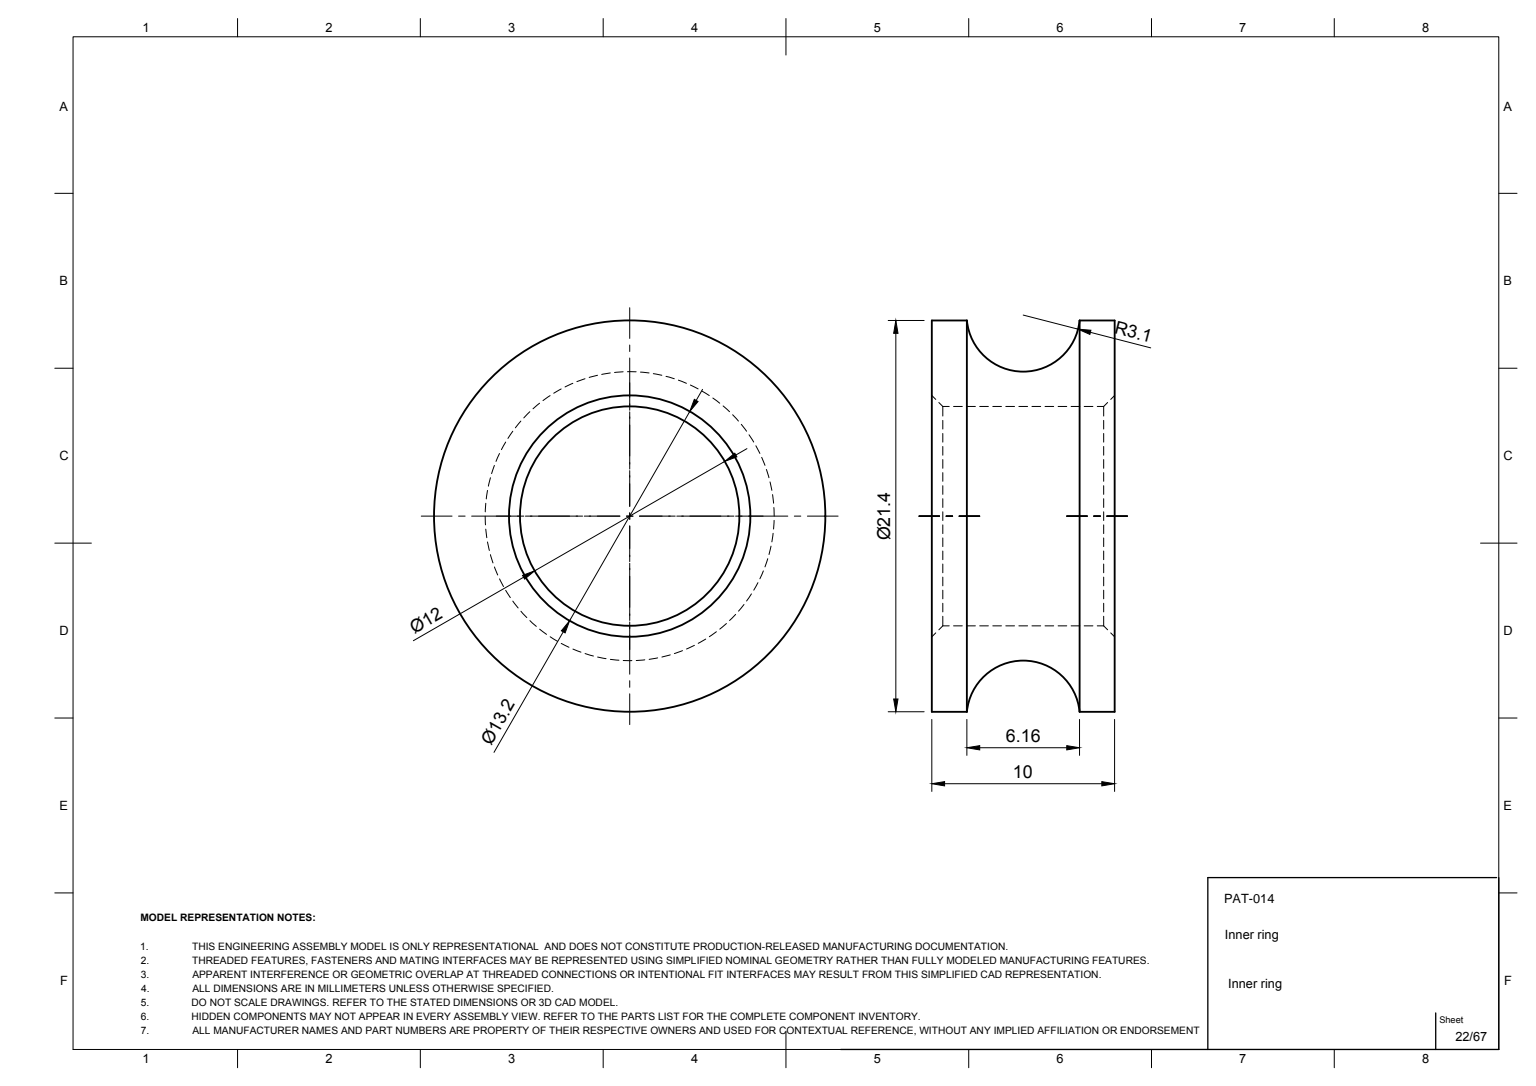
ISO-10303-21;
HEADER;
/* Generated by software containing ST-Developer
 * from STEP Tools, Inc. (www.steptools.com) 
 */

FILE_DESCRIPTION(
/* description */ ('Bin tilter linkage'),
/* implementation_level */ '2;1');

FILE_NAME(
/* name */ 'Inner ring.step',
/* time_stamp */ '2026-10-28T03:26:24-07:00',
/* author */ (''),
/* organization */ (''),
/* preprocessor_version */ 'ST-DEVELOPER v20.2',
/* originating_system */ 'Autodesk Translation Framework v15.17.0.0',
/* authorisation */ '');

FILE_SCHEMA (('AUTOMOTIVE_DESIGN { 1 0 10303 214 3 1 1 }'));
ENDSEC;

DATA;
#10=MECHANICAL_DESIGN_GEOMETRIC_PRESENTATION_REPRESENTATION('',(#934),#23728);
#627=TOROIDAL_SURFACE('',#14775,1.1,0.309556);
#636=CONICAL_SURFACE('',#14786,0.63,0.785398163397448);
#637=CONICAL_SURFACE('',#14793,0.63,0.785398163397448);
#722=SHAPE_REPRESENTATION_RELATIONSHIP('SRR','None',#24189,#828);
#828=ADVANCED_BREP_SHAPE_REPRESENTATION('',(#1047),#23689);
#934=STYLED_ITEM('',(#24765),#1047);
#1047=MANIFOLD_SOLID_BREP('Body1',#12465);
#1386=FACE_BOUND('',#3476,.T.);
#1387=FACE_BOUND('',#3479,.T.);
#1737=PLANE('',#14788);
#1738=PLANE('',#14791);
#2395=FACE_OUTER_BOUND('',#3471,.T.);
#2396=FACE_OUTER_BOUND('',#3472,.T.);
#2397=FACE_OUTER_BOUND('',#3473,.T.);
#2398=FACE_OUTER_BOUND('',#3474,.T.);
#2399=FACE_OUTER_BOUND('',#3475,.T.);
#2400=FACE_OUTER_BOUND('',#3477,.T.);
#2401=FACE_OUTER_BOUND('',#3478,.T.);
#2402=FACE_OUTER_BOUND('',#3480,.T.);
#3471=EDGE_LOOP('',(#10213,#10214,#10215,#10216,#10217,#10218));
#3472=EDGE_LOOP('',(#10219,#10220,#10221,#10222,#10223));
#3473=EDGE_LOOP('',(#10224,#10225,#10226,#10227));
#3474=EDGE_LOOP('',(#10228,#10229,#10230,#10231));
#3475=EDGE_LOOP('',(#10232));
#3476=EDGE_LOOP('',(#10233));
#3477=EDGE_LOOP('',(#10234,#10235,#10236,#10237,#10238));
#3478=EDGE_LOOP('',(#10239));
#3479=EDGE_LOOP('',(#10240));
#3480=EDGE_LOOP('',(#10241,#10242,#10243,#10244));
#4253=LINE('',#21872,#4928);
#4254=LINE('',#21878,#4929);
#4255=LINE('',#21882,#4930);
#4256=LINE('',#21888,#4931);
#4257=LINE('',#21893,#4932);
#4928=VECTOR('',#18090,1.070235);
#4929=VECTOR('',#18097,0.6);
#4930=VECTOR('',#18102,0.63);
#4931=VECTOR('',#18111,1.070235);
#4932=VECTOR('',#18118,0.63);
#5715=CIRCLE('',#14776,1.070235);
#5716=CIRCLE('',#14777,1.070235);
#5717=CIRCLE('',#14778,0.309556);
#5718=CIRCLE('',#14779,1.070235);
#5719=CIRCLE('',#14780,1.070235);
#5720=CIRCLE('',#14782,1.070235);
#5721=CIRCLE('',#14784,0.6);
#5722=CIRCLE('',#14785,0.6);
#5723=CIRCLE('',#14787,0.66);
#5724=CIRCLE('',#14790,1.070235);
#5725=CIRCLE('',#14792,0.66);
#6569=VERTEX_POINT('',#21861);
#6570=VERTEX_POINT('',#21862);
#6571=VERTEX_POINT('',#21865);
#6572=VERTEX_POINT('',#21867);
#6573=VERTEX_POINT('',#21871);
#6574=VERTEX_POINT('',#21875);
#6575=VERTEX_POINT('',#21877);
#6576=VERTEX_POINT('',#21881);
#6577=VERTEX_POINT('',#21886);
#6578=VERTEX_POINT('',#21890);
#7846=EDGE_CURVE('',#6569,#6570,#5715,.T.);
#7847=EDGE_CURVE('',#6570,#6569,#5716,.T.);
#7848=EDGE_CURVE('',#6570,#6571,#5717,.T.);
#7849=EDGE_CURVE('',#6572,#6571,#5718,.T.);
#7850=EDGE_CURVE('',#6571,#6572,#5719,.T.);
#7851=EDGE_CURVE('',#6572,#6573,#4253,.T.);
#7852=EDGE_CURVE('',#6573,#6573,#5720,.T.);
#7853=EDGE_CURVE('',#6574,#6574,#5721,.T.);
#7854=EDGE_CURVE('',#6574,#6575,#4254,.T.);
#7855=EDGE_CURVE('',#6575,#6575,#5722,.T.);
#7856=EDGE_CURVE('',#6575,#6576,#4255,.T.);
#7857=EDGE_CURVE('',#6576,#6576,#5723,.T.);
#7858=EDGE_CURVE('',#6577,#6577,#5724,.T.);
#7859=EDGE_CURVE('',#6577,#6569,#4256,.T.);
#7860=EDGE_CURVE('',#6578,#6578,#5725,.T.);
#7861=EDGE_CURVE('',#6578,#6574,#4257,.T.);
#10213=ORIENTED_EDGE('',*,*,#7846,.F.);
#10214=ORIENTED_EDGE('',*,*,#7847,.F.);
#10215=ORIENTED_EDGE('',*,*,#7848,.T.);
#10216=ORIENTED_EDGE('',*,*,#7849,.F.);
#10217=ORIENTED_EDGE('',*,*,#7850,.F.);
#10218=ORIENTED_EDGE('',*,*,#7848,.F.);
#10219=ORIENTED_EDGE('',*,*,#7849,.T.);
#10220=ORIENTED_EDGE('',*,*,#7850,.T.);
#10221=ORIENTED_EDGE('',*,*,#7851,.T.);
#10222=ORIENTED_EDGE('',*,*,#7852,.T.);
#10223=ORIENTED_EDGE('',*,*,#7851,.F.);
#10224=ORIENTED_EDGE('',*,*,#7853,.T.);
#10225=ORIENTED_EDGE('',*,*,#7854,.T.);
#10226=ORIENTED_EDGE('',*,*,#7855,.F.);
#10227=ORIENTED_EDGE('',*,*,#7854,.F.);
#10228=ORIENTED_EDGE('',*,*,#7855,.T.);
#10229=ORIENTED_EDGE('',*,*,#7856,.T.);
#10230=ORIENTED_EDGE('',*,*,#7857,.F.);
#10231=ORIENTED_EDGE('',*,*,#7856,.F.);
#10232=ORIENTED_EDGE('',*,*,#7852,.F.);
#10233=ORIENTED_EDGE('',*,*,#7857,.T.);
#10234=ORIENTED_EDGE('',*,*,#7858,.F.);
#10235=ORIENTED_EDGE('',*,*,#7859,.T.);
#10236=ORIENTED_EDGE('',*,*,#7846,.T.);
#10237=ORIENTED_EDGE('',*,*,#7847,.T.);
#10238=ORIENTED_EDGE('',*,*,#7859,.F.);
#10239=ORIENTED_EDGE('',*,*,#7858,.T.);
#10240=ORIENTED_EDGE('',*,*,#7860,.F.);
#10241=ORIENTED_EDGE('',*,*,#7860,.T.);
#10242=ORIENTED_EDGE('',*,*,#7861,.T.);
#10243=ORIENTED_EDGE('',*,*,#7853,.F.);
#10244=ORIENTED_EDGE('',*,*,#7861,.F.);
#11523=CYLINDRICAL_SURFACE('',#14781,1.070235);
#11524=CYLINDRICAL_SURFACE('',#14783,0.6);
#11525=CYLINDRICAL_SURFACE('',#14789,1.070235);
#12120=ADVANCED_FACE('',(#2395),#627,.F.);
#12121=ADVANCED_FACE('',(#2396),#11523,.T.);
#12122=ADVANCED_FACE('',(#2397),#11524,.F.);
#12123=ADVANCED_FACE('',(#2398),#636,.F.);
#12124=ADVANCED_FACE('',(#2399,#1386),#1737,.T.);
#12125=ADVANCED_FACE('',(#2400),#11525,.T.);
#12126=ADVANCED_FACE('',(#2401,#1387),#1738,.T.);
#12127=ADVANCED_FACE('',(#2402),#637,.F.);
#12465=CLOSED_SHELL('',(#12120,#12121,#12122,#12123,#12124,#12125,#12126,
#12127));
#14774=AXIS2_PLACEMENT_3D('',#21859,#18074,#18075);
#14775=AXIS2_PLACEMENT_3D('',#21860,#18076,#18077);
#14776=AXIS2_PLACEMENT_3D('',#21863,#18078,#18079);
#14777=AXIS2_PLACEMENT_3D('',#21864,#18080,#18081);
#14778=AXIS2_PLACEMENT_3D('',#21866,#18082,#18083);
#14779=AXIS2_PLACEMENT_3D('',#21868,#18084,#18085);
#14780=AXIS2_PLACEMENT_3D('',#21869,#18086,#18087);
#14781=AXIS2_PLACEMENT_3D('',#21870,#18088,#18089);
#14782=AXIS2_PLACEMENT_3D('',#21873,#18091,#18092);
#14783=AXIS2_PLACEMENT_3D('',#21874,#18093,#18094);
#14784=AXIS2_PLACEMENT_3D('',#21876,#18095,#18096);
#14785=AXIS2_PLACEMENT_3D('',#21879,#18098,#18099);
#14786=AXIS2_PLACEMENT_3D('',#21880,#18100,#18101);
#14787=AXIS2_PLACEMENT_3D('',#21883,#18103,#18104);
#14788=AXIS2_PLACEMENT_3D('',#21884,#18105,#18106);
#14789=AXIS2_PLACEMENT_3D('',#21885,#18107,#18108);
#14790=AXIS2_PLACEMENT_3D('',#21887,#18109,#18110);
#14791=AXIS2_PLACEMENT_3D('',#21889,#18112,#18113);
#14792=AXIS2_PLACEMENT_3D('',#21891,#18114,#18115);
#14793=AXIS2_PLACEMENT_3D('',#21892,#18116,#18117);
#18074=DIRECTION('axis',(0.,0.,1.));
#18075=DIRECTION('refdir',(1.,0.,0.));
#18076=DIRECTION('center_axis',(0.,-1.,0.));
#18077=DIRECTION('ref_axis',(0.,0.,-1.));
#18078=DIRECTION('center_axis',(0.,-1.,0.));
#18079=DIRECTION('ref_axis',(1.,0.,0.));
#18080=DIRECTION('center_axis',(0.,-1.,0.));
#18081=DIRECTION('ref_axis',(1.,0.,0.));
#18082=DIRECTION('center_axis',(1.,0.,1.22464679914735E-16));
#18083=DIRECTION('ref_axis',(-1.22464679914735E-16,0.,1.));
#18084=DIRECTION('center_axis',(0.,1.,0.));
#18085=DIRECTION('ref_axis',(1.,0.,0.));
#18086=DIRECTION('center_axis',(0.,1.,0.));
#18087=DIRECTION('ref_axis',(1.,0.,0.));
#18088=DIRECTION('center_axis',(0.,-1.,0.));
#18089=DIRECTION('ref_axis',(1.,0.,0.));
#18090=DIRECTION('',(0.,1.,0.));
#18091=DIRECTION('center_axis',(0.,-1.,0.));
#18092=DIRECTION('ref_axis',(1.,0.,0.));
#18093=DIRECTION('center_axis',(0.,-1.,0.));
#18094=DIRECTION('ref_axis',(1.,0.,0.));
#18095=DIRECTION('center_axis',(0.,-1.,0.));
#18096=DIRECTION('ref_axis',(1.,0.,0.));
#18097=DIRECTION('',(0.,1.,0.));
#18098=DIRECTION('center_axis',(0.,-1.,0.));
#18099=DIRECTION('ref_axis',(1.,0.,0.));
#18100=DIRECTION('center_axis',(0.,1.,0.));
#18101=DIRECTION('ref_axis',(1.,0.,0.));
#18102=DIRECTION('',(-0.707106781186548,0.707106781186547,-8.65956056235493E-17));
#18103=DIRECTION('center_axis',(0.,-1.,0.));
#18104=DIRECTION('ref_axis',(1.,0.,0.));
#18105=DIRECTION('center_axis',(0.,1.,0.));
#18106=DIRECTION('ref_axis',(0.,0.,1.));
#18107=DIRECTION('center_axis',(0.,-1.,0.));
#18108=DIRECTION('ref_axis',(1.,0.,0.));
#18109=DIRECTION('center_axis',(0.,-1.,0.));
#18110=DIRECTION('ref_axis',(1.,0.,0.));
#18111=DIRECTION('',(0.,1.,0.));
#18112=DIRECTION('center_axis',(0.,-1.,0.));
#18113=DIRECTION('ref_axis',(0.,0.,-1.));
#18114=DIRECTION('center_axis',(0.,-1.,0.));
#18115=DIRECTION('ref_axis',(1.,0.,0.));
#18116=DIRECTION('center_axis',(0.,-1.,0.));
#18117=DIRECTION('ref_axis',(1.,0.,0.));
#18118=DIRECTION('',(0.707106781186548,0.707106781186547,8.65956056235493E-17));
#21859=CARTESIAN_POINT('',(0.,0.,0.));
#21860=CARTESIAN_POINT('Origin',(0.,0.,0.));
#21861=CARTESIAN_POINT('',(-1.070235,-0.308121667383195,-1.31065986708547E-16));
#21862=CARTESIAN_POINT('',(-1.31065986708547E-16,-0.308121667383195,1.070235));
#21863=CARTESIAN_POINT('Origin',(0.,-0.308121667383195,0.));
#21864=CARTESIAN_POINT('Origin',(0.,-0.308121667383195,0.));
#21865=CARTESIAN_POINT('',(-1.31065986708547E-16,0.308121667383195,1.070235));
#21866=CARTESIAN_POINT('Origin',(-1.34711147906209E-16,0.,1.1));
#21867=CARTESIAN_POINT('',(-1.070235,0.308121667383195,1.31065986708547E-16));
#21868=CARTESIAN_POINT('Origin',(0.,0.308121667383195,0.));
#21869=CARTESIAN_POINT('Origin',(0.,0.308121667383195,0.));
#21870=CARTESIAN_POINT('Origin',(0.,0.,0.));
#21871=CARTESIAN_POINT('',(-1.070235,0.5,-1.31065986708547E-16));
#21872=CARTESIAN_POINT('',(-1.070235,0.,-1.31065986708547E-16));
#21873=CARTESIAN_POINT('Origin',(0.,0.5,0.));
#21874=CARTESIAN_POINT('Origin',(0.,0.,0.));
#21875=CARTESIAN_POINT('',(-0.6,-0.44,-7.34788079488412E-17));
#21876=CARTESIAN_POINT('Origin',(0.,-0.44,0.));
#21877=CARTESIAN_POINT('',(-0.6,0.44,-7.34788079488412E-17));
#21878=CARTESIAN_POINT('',(-0.6,0.,-7.34788079488412E-17));
#21879=CARTESIAN_POINT('Origin',(0.,0.44,0.));
#21880=CARTESIAN_POINT('Origin',(0.,0.47,0.));
#21881=CARTESIAN_POINT('',(-0.66,0.5,-8.08266887437253E-17));
#21882=CARTESIAN_POINT('',(-0.63,0.47,-7.71527483462832E-17));
#21883=CARTESIAN_POINT('Origin',(0.,0.5,0.));
#21884=CARTESIAN_POINT('Origin',(1.070235,0.5,0.));
#21885=CARTESIAN_POINT('Origin',(0.,0.,0.));
#21886=CARTESIAN_POINT('',(-1.070235,-0.5,-1.31065986708547E-16));
#21887=CARTESIAN_POINT('Origin',(0.,-0.5,0.));
#21888=CARTESIAN_POINT('',(-1.070235,0.,-1.31065986708547E-16));
#21889=CARTESIAN_POINT('Origin',(0.66,-0.5,0.));
#21890=CARTESIAN_POINT('',(-0.66,-0.5,-8.08266887437253E-17));
#21891=CARTESIAN_POINT('Origin',(0.,-0.5,0.));
#21892=CARTESIAN_POINT('Origin',(0.,-0.47,0.));
#21893=CARTESIAN_POINT('',(-0.63,-0.47,-7.71527483462832E-17));
#23572=UNCERTAINTY_MEASURE_WITH_UNIT(LENGTH_MEASURE(0.001),#23729,
'DISTANCE_ACCURACY_VALUE',
'Maximum model space distance between geometric entities at asserted c
onnectivities');
#23611=UNCERTAINTY_MEASURE_WITH_UNIT(LENGTH_MEASURE(0.001),#23729,
'DISTANCE_ACCURACY_VALUE',
'Maximum model space distance between geometric entities at asserted c
onnectivities');
#23689=(
GEOMETRIC_REPRESENTATION_CONTEXT(3)
GLOBAL_UNCERTAINTY_ASSIGNED_CONTEXT((#23572))
GLOBAL_UNIT_ASSIGNED_CONTEXT((#23729,#23731,#23732))
REPRESENTATION_CONTEXT('','3D')
);
#23728=(
GEOMETRIC_REPRESENTATION_CONTEXT(3)
GLOBAL_UNCERTAINTY_ASSIGNED_CONTEXT((#23611))
GLOBAL_UNIT_ASSIGNED_CONTEXT((#23729,#23731,#23732))
REPRESENTATION_CONTEXT('','3D')
);
#23729=(
LENGTH_UNIT()
NAMED_UNIT(*)
SI_UNIT(.CENTI.,.METRE.)
);
#23731=(
NAMED_UNIT(*)
PLANE_ANGLE_UNIT()
SI_UNIT($,.RADIAN.)
);
#23732=(
NAMED_UNIT(*)
SI_UNIT($,.STERADIAN.)
SOLID_ANGLE_UNIT()
);
#23810=SHAPE_DEFINITION_REPRESENTATION(#23926,#24189);
#23926=PRODUCT_DEFINITION_SHAPE('',$,#24306);
#24189=SHAPE_REPRESENTATION('',(#14774),#23689);
#24228=PRODUCT_DEFINITION_CONTEXT('part definition',#24578,'design');
#24306=PRODUCT_DEFINITION('Inner ring','Inner ring',#24422,#24228);
#24422=PRODUCT_DEFINITION_FORMATION('',$,#24657);
#24578=APPLICATION_CONTEXT(
'Core Data for Automotive Mechanical Design Process');
#24579=PRODUCT_CONTEXT('part definition',#24578,'mechanical');
#24657=PRODUCT('Inner ring','Inner ring','Inner ring',(#24579));
#24759=COLOUR_RGB('Grey',0.48,0.52,0.57);
#24760=FILL_AREA_STYLE_COLOUR('',#24759);
#24761=FILL_AREA_STYLE('',(#24760));
#24762=SURFACE_STYLE_FILL_AREA(#24761);
#24763=SURFACE_SIDE_STYLE('',(#24762));
#24764=SURFACE_STYLE_USAGE(.BOTH.,#24763);
#24765=PRESENTATION_STYLE_ASSIGNMENT((#24764));
ENDSEC;
END-ISO-10303-21;
